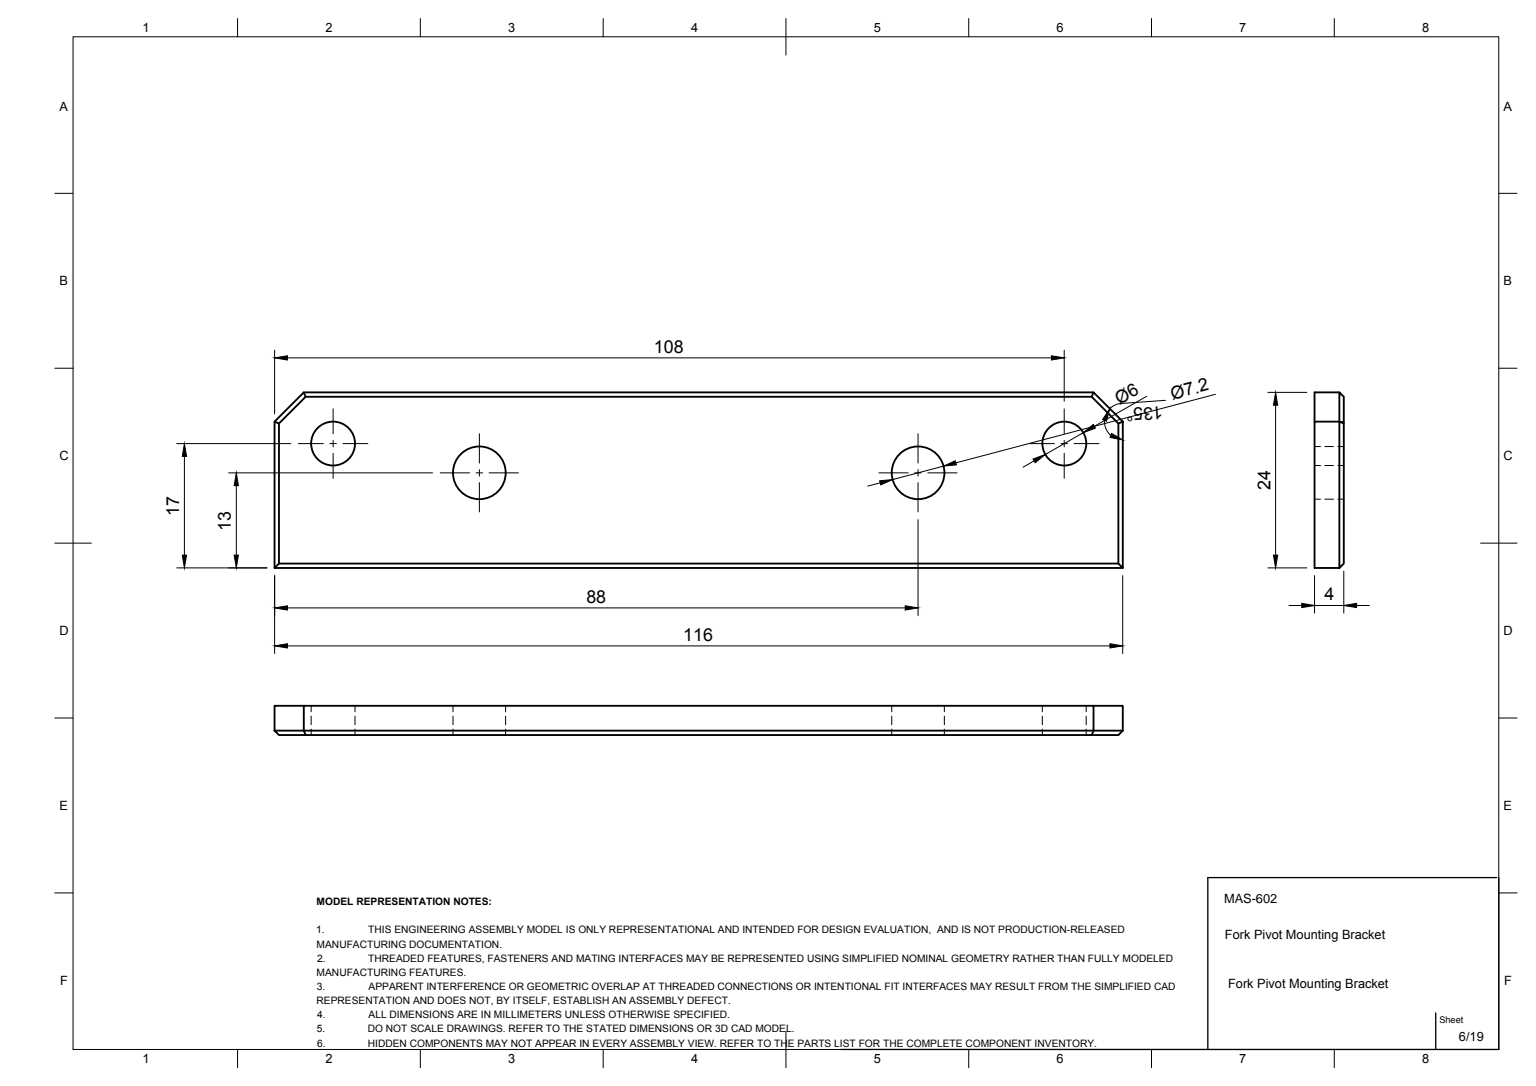
ISO-10303-21;
HEADER;
/* Generated by software containing ST-Developer
 * from STEP Tools, Inc. (www.steptools.com) 
 */

FILE_DESCRIPTION(
/* description */ (''),
/* implementation_level */ '2;1');

FILE_NAME(
/* name */ 'Fork Pivot Mounting Bracket.step',
/* time_stamp */ '2026-10-15T14:42:47-07:00',
/* author */ (''),
/* organization */ (''),
/* preprocessor_version */ 'ST-DEVELOPER v20.2',
/* originating_system */ 'Autodesk Translation Framework v15.15.0.0',
/* authorisation */ '');

FILE_SCHEMA (('AUTOMOTIVE_DESIGN { 1 0 10303 214 3 1 1 }'));
ENDSEC;

DATA;
#10=MECHANICAL_DESIGN_GEOMETRIC_PRESENTATION_REPRESENTATION('',(#237),#85789);
#201=SHAPE_REPRESENTATION_RELATIONSHIP('SRR','None',#85866,#219);
#219=ADVANCED_BREP_SHAPE_REPRESENTATION('',(#255),#85774);
#237=STYLED_ITEM('',(#85965),#255);
#255=MANIFOLD_SOLID_BREP('Body1',#9884);
#429=FACE_BOUND('',#3202,.T.);
#430=FACE_BOUND('',#3203,.T.);
#431=FACE_BOUND('',#3204,.T.);
#432=FACE_BOUND('',#3205,.T.);
#433=FACE_BOUND('',#3214,.T.);
#434=FACE_BOUND('',#3215,.T.);
#435=FACE_BOUND('',#3216,.T.);
#436=FACE_BOUND('',#3217,.T.);
#1066=PLANE('',#10454);
#1067=PLANE('',#10455);
#1068=PLANE('',#10456);
#1069=PLANE('',#10457);
#1070=PLANE('',#10458);
#1071=PLANE('',#10459);
#1072=PLANE('',#10460);
#1073=PLANE('',#10461);
#1074=PLANE('',#10462);
#1075=PLANE('',#10463);
#1076=PLANE('',#10476);
#1077=PLANE('',#10477);
#1078=PLANE('',#10478);
#1079=PLANE('',#10479);
#1435=LINE('',#23809,#1971);
#1436=LINE('',#23811,#1972);
#1437=LINE('',#23813,#1973);
#1438=LINE('',#23814,#1974);
#1439=LINE('',#23817,#1975);
#1440=LINE('',#23819,#1976);
#1441=LINE('',#23820,#1977);
#1442=LINE('',#23823,#1978);
#1443=LINE('',#23825,#1979);
#1444=LINE('',#23826,#1980);
#1445=LINE('',#23829,#1981);
#1446=LINE('',#23831,#1982);
#1447=LINE('',#23832,#1983);
#1448=LINE('',#23835,#1984);
#1449=LINE('',#23837,#1985);
#1450=LINE('',#23838,#1986);
#1451=LINE('',#23840,#1987);
#1452=LINE('',#23841,#1988);
#1453=LINE('',#23844,#1989);
#1454=LINE('',#23846,#1990);
#1455=LINE('',#23847,#1991);
#1456=LINE('',#23850,#1992);
#1457=LINE('',#23851,#1993);
#1458=LINE('',#23854,#1994);
#1459=LINE('',#23855,#1995);
#1460=LINE('',#23868,#1996);
#1461=LINE('',#23872,#1997);
#1462=LINE('',#23876,#1998);
#1463=LINE('',#23880,#1999);
#1464=LINE('',#23883,#2000);
#1465=LINE('',#23884,#2001);
#1466=LINE('',#23887,#2002);
#1467=LINE('',#23888,#2003);
#1468=LINE('',#23890,#2004);
#1971=VECTOR('',#11909,1.);
#1972=VECTOR('',#11910,1.);
#1973=VECTOR('',#11911,1.);
#1974=VECTOR('',#11912,1.);
#1975=VECTOR('',#11915,1.);
#1976=VECTOR('',#11916,1.);
#1977=VECTOR('',#11917,1.);
#1978=VECTOR('',#11920,1.);
#1979=VECTOR('',#11921,1.);
#1980=VECTOR('',#11922,1.);
#1981=VECTOR('',#11925,1.);
#1982=VECTOR('',#11926,1.);
#1983=VECTOR('',#11927,1.);
#1984=VECTOR('',#11930,1.);
#1985=VECTOR('',#11931,1.);
#1986=VECTOR('',#11932,1.);
#1987=VECTOR('',#11935,1.);
#1988=VECTOR('',#11936,1.);
#1989=VECTOR('',#11939,1.);
#1990=VECTOR('',#11940,1.);
#1991=VECTOR('',#11941,1.);
#1992=VECTOR('',#11944,1.);
#1993=VECTOR('',#11945,1.);
#1994=VECTOR('',#11948,1.);
#1995=VECTOR('',#11949,1.);
#1996=VECTOR('',#11964,0.36);
#1997=VECTOR('',#11969,0.3);
#1998=VECTOR('',#11974,0.3);
#1999=VECTOR('',#11979,0.36);
#2000=VECTOR('',#11982,1.);
#2001=VECTOR('',#11983,1.);
#2002=VECTOR('',#11986,1.);
#2003=VECTOR('',#11987,1.);
#2004=VECTOR('',#11990,1.);
#2322=CYLINDRICAL_SURFACE('',#10468,0.36);
#2323=CYLINDRICAL_SURFACE('',#10470,0.3);
#2324=CYLINDRICAL_SURFACE('',#10472,0.3);
#2325=CYLINDRICAL_SURFACE('',#10474,0.36);
#2648=FACE_OUTER_BOUND('',#3192,.T.);
#2649=FACE_OUTER_BOUND('',#3193,.T.);
#2650=FACE_OUTER_BOUND('',#3194,.T.);
#2651=FACE_OUTER_BOUND('',#3195,.T.);
#2652=FACE_OUTER_BOUND('',#3196,.T.);
#2653=FACE_OUTER_BOUND('',#3197,.T.);
#2654=FACE_OUTER_BOUND('',#3198,.T.);
#2655=FACE_OUTER_BOUND('',#3199,.T.);
#2656=FACE_OUTER_BOUND('',#3200,.T.);
#2657=FACE_OUTER_BOUND('',#3201,.T.);
#2658=FACE_OUTER_BOUND('',#3206,.T.);
#2659=FACE_OUTER_BOUND('',#3207,.T.);
#2660=FACE_OUTER_BOUND('',#3208,.T.);
#2661=FACE_OUTER_BOUND('',#3209,.T.);
#2662=FACE_OUTER_BOUND('',#3210,.T.);
#2663=FACE_OUTER_BOUND('',#3211,.T.);
#2664=FACE_OUTER_BOUND('',#3212,.T.);
#2665=FACE_OUTER_BOUND('',#3213,.T.);
#3192=EDGE_LOOP('',(#7641,#7642,#7643,#7644));
#3193=EDGE_LOOP('',(#7645,#7646,#7647,#7648));
#3194=EDGE_LOOP('',(#7649,#7650,#7651,#7652));
#3195=EDGE_LOOP('',(#7653,#7654,#7655,#7656));
#3196=EDGE_LOOP('',(#7657,#7658,#7659,#7660));
#3197=EDGE_LOOP('',(#7661,#7662,#7663,#7664));
#3198=EDGE_LOOP('',(#7665,#7666,#7667,#7668));
#3199=EDGE_LOOP('',(#7669,#7670,#7671,#7672));
#3200=EDGE_LOOP('',(#7673,#7674,#7675,#7676));
#3201=EDGE_LOOP('',(#7677,#7678,#7679,#7680,#7681,#7682));
#3202=EDGE_LOOP('',(#7683));
#3203=EDGE_LOOP('',(#7684));
#3204=EDGE_LOOP('',(#7685));
#3205=EDGE_LOOP('',(#7686));
#3206=EDGE_LOOP('',(#7687,#7688,#7689,#7690));
#3207=EDGE_LOOP('',(#7691,#7692,#7693,#7694));
#3208=EDGE_LOOP('',(#7695,#7696,#7697,#7698));
#3209=EDGE_LOOP('',(#7699,#7700,#7701,#7702));
#3210=EDGE_LOOP('',(#7703,#7704,#7705,#7706));
#3211=EDGE_LOOP('',(#7707,#7708,#7709,#7710));
#3212=EDGE_LOOP('',(#7711,#7712,#7713,#7714));
#3213=EDGE_LOOP('',(#7715,#7716,#7717,#7718,#7719,#7720));
#3214=EDGE_LOOP('',(#7721));
#3215=EDGE_LOOP('',(#7722));
#3216=EDGE_LOOP('',(#7723));
#3217=EDGE_LOOP('',(#7724));
#3684=CIRCLE('',#10464,0.36);
#3685=CIRCLE('',#10465,0.3);
#3686=CIRCLE('',#10466,0.3);
#3687=CIRCLE('',#10467,0.36);
#3688=CIRCLE('',#10469,0.36);
#3689=CIRCLE('',#10471,0.3);
#3690=CIRCLE('',#10473,0.3);
#3691=CIRCLE('',#10475,0.36);
#4275=VERTEX_POINT('',#23807);
#4276=VERTEX_POINT('',#23808);
#4277=VERTEX_POINT('',#23810);
#4278=VERTEX_POINT('',#23812);
#4279=VERTEX_POINT('',#23816);
#4280=VERTEX_POINT('',#23818);
#4281=VERTEX_POINT('',#23822);
#4282=VERTEX_POINT('',#23824);
#4283=VERTEX_POINT('',#23828);
#4284=VERTEX_POINT('',#23830);
#4285=VERTEX_POINT('',#23834);
#4286=VERTEX_POINT('',#23836);
#4287=VERTEX_POINT('',#23843);
#4288=VERTEX_POINT('',#23845);
#4289=VERTEX_POINT('',#23849);
#4290=VERTEX_POINT('',#23853);
#4291=VERTEX_POINT('',#23857);
#4292=VERTEX_POINT('',#23859);
#4293=VERTEX_POINT('',#23861);
#4294=VERTEX_POINT('',#23863);
#4295=VERTEX_POINT('',#23866);
#4296=VERTEX_POINT('',#23870);
#4297=VERTEX_POINT('',#23874);
#4298=VERTEX_POINT('',#23878);
#4299=VERTEX_POINT('',#23882);
#4300=VERTEX_POINT('',#23886);
#5548=EDGE_CURVE('',#4275,#4276,#1435,.T.);
#5549=EDGE_CURVE('',#4276,#4277,#1436,.T.);
#5550=EDGE_CURVE('',#4277,#4278,#1437,.T.);
#5551=EDGE_CURVE('',#4275,#4278,#1438,.T.);
#5552=EDGE_CURVE('',#4276,#4279,#1439,.T.);
#5553=EDGE_CURVE('',#4279,#4280,#1440,.T.);
#5554=EDGE_CURVE('',#4280,#4277,#1441,.T.);
#5555=EDGE_CURVE('',#4279,#4281,#1442,.T.);
#5556=EDGE_CURVE('',#4281,#4282,#1443,.T.);
#5557=EDGE_CURVE('',#4282,#4280,#1444,.T.);
#5558=EDGE_CURVE('',#4281,#4283,#1445,.T.);
#5559=EDGE_CURVE('',#4283,#4284,#1446,.T.);
#5560=EDGE_CURVE('',#4284,#4282,#1447,.T.);
#5561=EDGE_CURVE('',#4285,#4284,#1448,.T.);
#5562=EDGE_CURVE('',#4283,#4286,#1449,.T.);
#5563=EDGE_CURVE('',#4286,#4285,#1450,.T.);
#5564=EDGE_CURVE('',#4278,#4285,#1451,.T.);
#5565=EDGE_CURVE('',#4286,#4275,#1452,.T.);
#5566=EDGE_CURVE('',#4287,#4285,#1453,.T.);
#5567=EDGE_CURVE('',#4287,#4288,#1454,.T.);
#5568=EDGE_CURVE('',#4288,#4284,#1455,.T.);
#5569=EDGE_CURVE('',#4289,#4278,#1456,.T.);
#5570=EDGE_CURVE('',#4289,#4287,#1457,.T.);
#5571=EDGE_CURVE('',#4290,#4277,#1458,.T.);
#5572=EDGE_CURVE('',#4290,#4289,#1459,.T.);
#5573=EDGE_CURVE('',#4291,#4291,#3684,.T.);
#5574=EDGE_CURVE('',#4292,#4292,#3685,.T.);
#5575=EDGE_CURVE('',#4293,#4293,#3686,.T.);
#5576=EDGE_CURVE('',#4294,#4294,#3687,.T.);
#5577=EDGE_CURVE('',#4295,#4295,#3688,.T.);
#5578=EDGE_CURVE('',#4295,#4294,#1460,.T.);
#5579=EDGE_CURVE('',#4296,#4296,#3689,.T.);
#5580=EDGE_CURVE('',#4296,#4293,#1461,.T.);
#5581=EDGE_CURVE('',#4297,#4297,#3690,.T.);
#5582=EDGE_CURVE('',#4297,#4292,#1462,.T.);
#5583=EDGE_CURVE('',#4298,#4298,#3691,.T.);
#5584=EDGE_CURVE('',#4298,#4291,#1463,.T.);
#5585=EDGE_CURVE('',#4299,#4280,#1464,.T.);
#5586=EDGE_CURVE('',#4299,#4290,#1465,.T.);
#5587=EDGE_CURVE('',#4300,#4282,#1466,.T.);
#5588=EDGE_CURVE('',#4300,#4299,#1467,.T.);
#5589=EDGE_CURVE('',#4288,#4300,#1468,.T.);
#7641=ORIENTED_EDGE('',*,*,#5548,.T.);
#7642=ORIENTED_EDGE('',*,*,#5549,.T.);
#7643=ORIENTED_EDGE('',*,*,#5550,.T.);
#7644=ORIENTED_EDGE('',*,*,#5551,.F.);
#7645=ORIENTED_EDGE('',*,*,#5552,.T.);
#7646=ORIENTED_EDGE('',*,*,#5553,.T.);
#7647=ORIENTED_EDGE('',*,*,#5554,.T.);
#7648=ORIENTED_EDGE('',*,*,#5549,.F.);
#7649=ORIENTED_EDGE('',*,*,#5555,.T.);
#7650=ORIENTED_EDGE('',*,*,#5556,.T.);
#7651=ORIENTED_EDGE('',*,*,#5557,.T.);
#7652=ORIENTED_EDGE('',*,*,#5553,.F.);
#7653=ORIENTED_EDGE('',*,*,#5558,.T.);
#7654=ORIENTED_EDGE('',*,*,#5559,.T.);
#7655=ORIENTED_EDGE('',*,*,#5560,.T.);
#7656=ORIENTED_EDGE('',*,*,#5556,.F.);
#7657=ORIENTED_EDGE('',*,*,#5561,.T.);
#7658=ORIENTED_EDGE('',*,*,#5559,.F.);
#7659=ORIENTED_EDGE('',*,*,#5562,.T.);
#7660=ORIENTED_EDGE('',*,*,#5563,.T.);
#7661=ORIENTED_EDGE('',*,*,#5564,.T.);
#7662=ORIENTED_EDGE('',*,*,#5563,.F.);
#7663=ORIENTED_EDGE('',*,*,#5565,.T.);
#7664=ORIENTED_EDGE('',*,*,#5551,.T.);
#7665=ORIENTED_EDGE('',*,*,#5561,.F.);
#7666=ORIENTED_EDGE('',*,*,#5566,.F.);
#7667=ORIENTED_EDGE('',*,*,#5567,.T.);
#7668=ORIENTED_EDGE('',*,*,#5568,.T.);
#7669=ORIENTED_EDGE('',*,*,#5564,.F.);
#7670=ORIENTED_EDGE('',*,*,#5569,.F.);
#7671=ORIENTED_EDGE('',*,*,#5570,.T.);
#7672=ORIENTED_EDGE('',*,*,#5566,.T.);
#7673=ORIENTED_EDGE('',*,*,#5550,.F.);
#7674=ORIENTED_EDGE('',*,*,#5571,.F.);
#7675=ORIENTED_EDGE('',*,*,#5572,.T.);
#7676=ORIENTED_EDGE('',*,*,#5569,.T.);
#7677=ORIENTED_EDGE('',*,*,#5548,.F.);
#7678=ORIENTED_EDGE('',*,*,#5565,.F.);
#7679=ORIENTED_EDGE('',*,*,#5562,.F.);
#7680=ORIENTED_EDGE('',*,*,#5558,.F.);
#7681=ORIENTED_EDGE('',*,*,#5555,.F.);
#7682=ORIENTED_EDGE('',*,*,#5552,.F.);
#7683=ORIENTED_EDGE('',*,*,#5573,.T.);
#7684=ORIENTED_EDGE('',*,*,#5574,.T.);
#7685=ORIENTED_EDGE('',*,*,#5575,.T.);
#7686=ORIENTED_EDGE('',*,*,#5576,.T.);
#7687=ORIENTED_EDGE('',*,*,#5577,.F.);
#7688=ORIENTED_EDGE('',*,*,#5578,.T.);
#7689=ORIENTED_EDGE('',*,*,#5576,.F.);
#7690=ORIENTED_EDGE('',*,*,#5578,.F.);
#7691=ORIENTED_EDGE('',*,*,#5579,.F.);
#7692=ORIENTED_EDGE('',*,*,#5580,.T.);
#7693=ORIENTED_EDGE('',*,*,#5575,.F.);
#7694=ORIENTED_EDGE('',*,*,#5580,.F.);
#7695=ORIENTED_EDGE('',*,*,#5581,.F.);
#7696=ORIENTED_EDGE('',*,*,#5582,.T.);
#7697=ORIENTED_EDGE('',*,*,#5574,.F.);
#7698=ORIENTED_EDGE('',*,*,#5582,.F.);
#7699=ORIENTED_EDGE('',*,*,#5583,.F.);
#7700=ORIENTED_EDGE('',*,*,#5584,.T.);
#7701=ORIENTED_EDGE('',*,*,#5573,.F.);
#7702=ORIENTED_EDGE('',*,*,#5584,.F.);
#7703=ORIENTED_EDGE('',*,*,#5554,.F.);
#7704=ORIENTED_EDGE('',*,*,#5585,.F.);
#7705=ORIENTED_EDGE('',*,*,#5586,.T.);
#7706=ORIENTED_EDGE('',*,*,#5571,.T.);
#7707=ORIENTED_EDGE('',*,*,#5557,.F.);
#7708=ORIENTED_EDGE('',*,*,#5587,.F.);
#7709=ORIENTED_EDGE('',*,*,#5588,.T.);
#7710=ORIENTED_EDGE('',*,*,#5585,.T.);
#7711=ORIENTED_EDGE('',*,*,#5560,.F.);
#7712=ORIENTED_EDGE('',*,*,#5568,.F.);
#7713=ORIENTED_EDGE('',*,*,#5589,.T.);
#7714=ORIENTED_EDGE('',*,*,#5587,.T.);
#7715=ORIENTED_EDGE('',*,*,#5589,.F.);
#7716=ORIENTED_EDGE('',*,*,#5567,.F.);
#7717=ORIENTED_EDGE('',*,*,#5570,.F.);
#7718=ORIENTED_EDGE('',*,*,#5572,.F.);
#7719=ORIENTED_EDGE('',*,*,#5586,.F.);
#7720=ORIENTED_EDGE('',*,*,#5588,.F.);
#7721=ORIENTED_EDGE('',*,*,#5577,.T.);
#7722=ORIENTED_EDGE('',*,*,#5579,.T.);
#7723=ORIENTED_EDGE('',*,*,#5581,.T.);
#7724=ORIENTED_EDGE('',*,*,#5583,.T.);
#9626=ADVANCED_FACE('',(#2648),#1066,.T.);
#9627=ADVANCED_FACE('',(#2649),#1067,.T.);
#9628=ADVANCED_FACE('',(#2650),#1068,.T.);
#9629=ADVANCED_FACE('',(#2651),#1069,.T.);
#9630=ADVANCED_FACE('',(#2652),#1070,.T.);
#9631=ADVANCED_FACE('',(#2653),#1071,.T.);
#9632=ADVANCED_FACE('',(#2654),#1072,.T.);
#9633=ADVANCED_FACE('',(#2655),#1073,.T.);
#9634=ADVANCED_FACE('',(#2656),#1074,.T.);
#9635=ADVANCED_FACE('',(#2657,#429,#430,#431,#432),#1075,.T.);
#9636=ADVANCED_FACE('',(#2658),#2322,.F.);
#9637=ADVANCED_FACE('',(#2659),#2323,.F.);
#9638=ADVANCED_FACE('',(#2660),#2324,.F.);
#9639=ADVANCED_FACE('',(#2661),#2325,.F.);
#9640=ADVANCED_FACE('',(#2662),#1076,.T.);
#9641=ADVANCED_FACE('',(#2663),#1077,.T.);
#9642=ADVANCED_FACE('',(#2664),#1078,.T.);
#9643=ADVANCED_FACE('',(#2665,#433,#434,#435,#436),#1079,.T.);
#9884=CLOSED_SHELL('',(#9626,#9627,#9628,#9629,#9630,#9631,#9632,#9633,
#9634,#9635,#9636,#9637,#9638,#9639,#9640,#9641,#9642,#9643));
#10453=AXIS2_PLACEMENT_3D('',#23805,#11905,#11906);
#10454=AXIS2_PLACEMENT_3D('',#23806,#11907,#11908);
#10455=AXIS2_PLACEMENT_3D('',#23815,#11913,#11914);
#10456=AXIS2_PLACEMENT_3D('',#23821,#11918,#11919);
#10457=AXIS2_PLACEMENT_3D('',#23827,#11923,#11924);
#10458=AXIS2_PLACEMENT_3D('',#23833,#11928,#11929);
#10459=AXIS2_PLACEMENT_3D('',#23839,#11933,#11934);
#10460=AXIS2_PLACEMENT_3D('',#23842,#11937,#11938);
#10461=AXIS2_PLACEMENT_3D('',#23848,#11942,#11943);
#10462=AXIS2_PLACEMENT_3D('',#23852,#11946,#11947);
#10463=AXIS2_PLACEMENT_3D('',#23856,#11950,#11951);
#10464=AXIS2_PLACEMENT_3D('',#23858,#11952,#11953);
#10465=AXIS2_PLACEMENT_3D('',#23860,#11954,#11955);
#10466=AXIS2_PLACEMENT_3D('',#23862,#11956,#11957);
#10467=AXIS2_PLACEMENT_3D('',#23864,#11958,#11959);
#10468=AXIS2_PLACEMENT_3D('',#23865,#11960,#11961);
#10469=AXIS2_PLACEMENT_3D('',#23867,#11962,#11963);
#10470=AXIS2_PLACEMENT_3D('',#23869,#11965,#11966);
#10471=AXIS2_PLACEMENT_3D('',#23871,#11967,#11968);
#10472=AXIS2_PLACEMENT_3D('',#23873,#11970,#11971);
#10473=AXIS2_PLACEMENT_3D('',#23875,#11972,#11973);
#10474=AXIS2_PLACEMENT_3D('',#23877,#11975,#11976);
#10475=AXIS2_PLACEMENT_3D('',#23879,#11977,#11978);
#10476=AXIS2_PLACEMENT_3D('',#23881,#11980,#11981);
#10477=AXIS2_PLACEMENT_3D('',#23885,#11984,#11985);
#10478=AXIS2_PLACEMENT_3D('',#23889,#11988,#11989);
#10479=AXIS2_PLACEMENT_3D('',#23891,#11991,#11992);
#11905=DIRECTION('axis',(0.,0.,1.));
#11906=DIRECTION('refdir',(1.,0.,0.));
#11907=DIRECTION('center_axis',(0.70710678118655,-0.707106781186545,0.));
#11908=DIRECTION('ref_axis',(0.,0.,-1.));
#11909=DIRECTION('',(0.,0.,-1.));
#11910=DIRECTION('',(0.577350269189622,0.577350269189625,-0.57735026918963));
#11911=DIRECTION('',(0.,0.,1.));
#11912=DIRECTION('',(0.678598344545843,0.678598344545847,0.281084637714829));
#11913=DIRECTION('center_axis',(0.,-0.70710678118655,-0.707106781186545));
#11914=DIRECTION('ref_axis',(-1.,0.,0.));
#11915=DIRECTION('',(-1.,0.,0.));
#11916=DIRECTION('',(-0.577350269189622,0.577350269189625,-0.57735026918963));
#11917=DIRECTION('',(1.,0.,0.));
#11918=DIRECTION('center_axis',(-0.70710678118655,-0.707106781186545,0.));
#11919=DIRECTION('ref_axis',(0.,0.,1.));
#11920=DIRECTION('',(0.,0.,1.));
#11921=DIRECTION('',(-0.678598344545839,0.678598344545844,0.281084637714847));
#11922=DIRECTION('',(0.,0.,-1.));
#11923=DIRECTION('center_axis',(-0.499999999999994,-0.707106781186556,0.499999999999993));
#11924=DIRECTION('ref_axis',(0.707106781186547,-1.66533453693739E-16,0.707106781186548));
#11925=DIRECTION('',(0.707106781186547,0.,0.707106781186548));
#11926=DIRECTION('',(-0.281084637714836,0.678598344545841,0.678598344545847));
#11927=DIRECTION('',(-0.707106781186547,0.,-0.707106781186548));
#11928=DIRECTION('center_axis',(0.,-0.70710678118655,0.707106781186545));
#11929=DIRECTION('ref_axis',(1.,0.,0.));
#11930=DIRECTION('',(-1.,0.,0.));
#11931=DIRECTION('',(1.,0.,0.));
#11932=DIRECTION('',(0.281084637714827,0.678598344545843,0.678598344545848));
#11933=DIRECTION('center_axis',(0.499999999999997,-0.707106781186553,0.499999999999996));
#11934=DIRECTION('ref_axis',(0.707106781186547,1.66533453693763E-16,-0.707106781186548));
#11935=DIRECTION('',(-0.707106781186547,0.,0.707106781186548));
#11936=DIRECTION('',(0.707106781186547,0.,-0.707106781186548));
#11937=DIRECTION('center_axis',(0.,0.,1.));
#11938=DIRECTION('ref_axis',(-1.,0.,0.));
#11939=DIRECTION('',(0.,-1.,0.));
#11940=DIRECTION('',(-1.,0.,0.));
#11941=DIRECTION('',(0.,-1.,0.));
#11942=DIRECTION('center_axis',(0.707106781186548,0.,0.707106781186547));
#11943=DIRECTION('ref_axis',(-0.707106781186547,0.,0.707106781186548));
#11944=DIRECTION('',(0.,-1.,0.));
#11945=DIRECTION('',(-0.707106781186547,0.,0.707106781186548));
#11946=DIRECTION('center_axis',(1.,0.,0.));
#11947=DIRECTION('ref_axis',(0.,0.,1.));
#11948=DIRECTION('',(0.,-1.,0.));
#11949=DIRECTION('',(0.,0.,1.));
#11950=DIRECTION('center_axis',(0.,-1.,0.));
#11951=DIRECTION('ref_axis',(0.,0.,-1.));
#11952=DIRECTION('center_axis',(0.,1.,0.));
#11953=DIRECTION('ref_axis',(1.,0.,0.));
#11954=DIRECTION('center_axis',(0.,1.,0.));
#11955=DIRECTION('ref_axis',(1.,0.,0.));
#11956=DIRECTION('center_axis',(0.,1.,0.));
#11957=DIRECTION('ref_axis',(1.,0.,0.));
#11958=DIRECTION('center_axis',(0.,1.,0.));
#11959=DIRECTION('ref_axis',(1.,0.,0.));
#11960=DIRECTION('center_axis',(0.,-1.,0.));
#11961=DIRECTION('ref_axis',(1.,0.,0.));
#11962=DIRECTION('center_axis',(0.,-1.,0.));
#11963=DIRECTION('ref_axis',(1.,0.,0.));
#11964=DIRECTION('',(0.,-1.,0.));
#11965=DIRECTION('center_axis',(0.,-1.,0.));
#11966=DIRECTION('ref_axis',(1.,0.,0.));
#11967=DIRECTION('center_axis',(0.,-1.,0.));
#11968=DIRECTION('ref_axis',(1.,0.,0.));
#11969=DIRECTION('',(0.,-1.,0.));
#11970=DIRECTION('center_axis',(0.,-1.,0.));
#11971=DIRECTION('ref_axis',(1.,0.,0.));
#11972=DIRECTION('center_axis',(0.,-1.,0.));
#11973=DIRECTION('ref_axis',(1.,0.,0.));
#11974=DIRECTION('',(0.,-1.,0.));
#11975=DIRECTION('center_axis',(0.,-1.,0.));
#11976=DIRECTION('ref_axis',(1.,0.,0.));
#11977=DIRECTION('center_axis',(0.,-1.,0.));
#11978=DIRECTION('ref_axis',(1.,0.,0.));
#11979=DIRECTION('',(0.,-1.,0.));
#11980=DIRECTION('center_axis',(0.,0.,-1.));
#11981=DIRECTION('ref_axis',(1.,0.,0.));
#11982=DIRECTION('',(0.,-1.,0.));
#11983=DIRECTION('',(1.,0.,0.));
#11984=DIRECTION('center_axis',(-1.,0.,0.));
#11985=DIRECTION('ref_axis',(0.,0.,-1.));
#11986=DIRECTION('',(0.,-1.,0.));
#11987=DIRECTION('',(0.,0.,-1.));
#11988=DIRECTION('center_axis',(-0.707106781186548,0.,0.707106781186547));
#11989=DIRECTION('ref_axis',(-0.707106781186547,0.,-0.707106781186548));
#11990=DIRECTION('',(-0.707106781186547,0.,-0.707106781186548));
#11991=DIRECTION('center_axis',(0.,1.,0.));
#11992=DIRECTION('ref_axis',(1.,0.,0.));
#23805=CARTESIAN_POINT('',(0.,0.,0.));
#23806=CARTESIAN_POINT('Origin',(5.77,-0.37,11.));
#23807=CARTESIAN_POINT('',(5.74,-0.4,12.3751471862576));
#23808=CARTESIAN_POINT('',(5.74,-0.4,10.46));
#23809=CARTESIAN_POINT('',(5.74,-0.4,11.));
#23810=CARTESIAN_POINT('',(5.8,-0.34,10.4));
#23811=CARTESIAN_POINT('',(5.74,-0.4,10.46));
#23812=CARTESIAN_POINT('',(5.8,-0.34,12.4));
#23813=CARTESIAN_POINT('',(5.8,-0.34,11.));
#23814=CARTESIAN_POINT('',(5.74,-0.4,12.3751471862576));
#23815=CARTESIAN_POINT('Origin',(-2.9,-0.37,10.43));
#23816=CARTESIAN_POINT('',(-5.74,-0.4,10.46));
#23817=CARTESIAN_POINT('',(-2.9,-0.4,10.46));
#23818=CARTESIAN_POINT('',(-5.8,-0.34,10.4));
#23819=CARTESIAN_POINT('',(-5.74,-0.4,10.46));
#23820=CARTESIAN_POINT('',(-2.9,-0.34,10.4));
#23821=CARTESIAN_POINT('Origin',(-5.77,-0.37,12.));
#23822=CARTESIAN_POINT('',(-5.74,-0.4,12.3751471862576));
#23823=CARTESIAN_POINT('',(-5.74,-0.4,12.));
#23824=CARTESIAN_POINT('',(-5.8,-0.34,12.4));
#23825=CARTESIAN_POINT('',(-5.74,-0.4,12.3751471862576));
#23826=CARTESIAN_POINT('',(-5.8,-0.34,12.));
#23827=CARTESIAN_POINT('Origin',(-4.32878679656441,-0.37,13.8287867965644));
#23828=CARTESIAN_POINT('',(-5.37514718625761,-0.4,12.74));
#23829=CARTESIAN_POINT('',(-4.30757359312881,-0.4,13.8075735931288));
#23830=CARTESIAN_POINT('',(-5.4,-0.34,12.8));
#23831=CARTESIAN_POINT('',(-5.37514718625761,-0.4,12.74));
#23832=CARTESIAN_POINT('',(-4.35,-0.34,13.85));
#23833=CARTESIAN_POINT('Origin',(2.7,-0.37,12.77));
#23834=CARTESIAN_POINT('',(5.4,-0.34,12.8));
#23835=CARTESIAN_POINT('',(2.7,-0.34,12.8));
#23836=CARTESIAN_POINT('',(5.37514718625761,-0.4,12.74));
#23837=CARTESIAN_POINT('',(2.7,-0.4,12.74));
#23838=CARTESIAN_POINT('',(5.37514718625761,-0.4,12.74));
#23839=CARTESIAN_POINT('Origin',(4.52878679656441,-0.37,13.6287867965644));
#23840=CARTESIAN_POINT('',(4.55,-0.34,13.65));
#23841=CARTESIAN_POINT('',(4.50757359312881,-0.4,13.6075735931288));
#23842=CARTESIAN_POINT('Origin',(5.4,0.,12.8));
#23843=CARTESIAN_POINT('',(5.4,0.,12.8));
#23844=CARTESIAN_POINT('',(5.4,0.,12.8));
#23845=CARTESIAN_POINT('',(-5.4,0.,12.8));
#23846=CARTESIAN_POINT('',(5.4,0.,12.8));
#23847=CARTESIAN_POINT('',(-5.4,0.,12.8));
#23848=CARTESIAN_POINT('Origin',(5.8,0.,12.4));
#23849=CARTESIAN_POINT('',(5.8,0.,12.4));
#23850=CARTESIAN_POINT('',(5.8,0.,12.4));
#23851=CARTESIAN_POINT('',(5.8,0.,12.4));
#23852=CARTESIAN_POINT('Origin',(5.8,0.,10.4));
#23853=CARTESIAN_POINT('',(5.8,0.,10.4));
#23854=CARTESIAN_POINT('',(5.8,0.,10.4));
#23855=CARTESIAN_POINT('',(5.8,0.,10.4));
#23856=CARTESIAN_POINT('Origin',(0.,-0.4,11.6));
#23857=CARTESIAN_POINT('',(-3.36,-0.4,11.7));
#23858=CARTESIAN_POINT('Origin',(-3.,-0.4,11.7));
#23859=CARTESIAN_POINT('',(4.7,-0.4,12.1));
#23860=CARTESIAN_POINT('Origin',(5.,-0.4,12.1));
#23861=CARTESIAN_POINT('',(-5.3,-0.4,12.1));
#23862=CARTESIAN_POINT('Origin',(-5.,-0.4,12.1));
#23863=CARTESIAN_POINT('',(2.64,-0.4,11.7));
#23864=CARTESIAN_POINT('Origin',(3.,-0.4,11.7));
#23865=CARTESIAN_POINT('Origin',(3.,0.,11.7));
#23866=CARTESIAN_POINT('',(2.64,0.,11.7));
#23867=CARTESIAN_POINT('Origin',(3.,0.,11.7));
#23868=CARTESIAN_POINT('',(2.64,0.,11.7));
#23869=CARTESIAN_POINT('Origin',(-5.,0.,12.1));
#23870=CARTESIAN_POINT('',(-5.3,0.,12.1));
#23871=CARTESIAN_POINT('Origin',(-5.,0.,12.1));
#23872=CARTESIAN_POINT('',(-5.3,0.,12.1));
#23873=CARTESIAN_POINT('Origin',(5.,0.,12.1));
#23874=CARTESIAN_POINT('',(4.7,0.,12.1));
#23875=CARTESIAN_POINT('Origin',(5.,0.,12.1));
#23876=CARTESIAN_POINT('',(4.7,0.,12.1));
#23877=CARTESIAN_POINT('Origin',(-3.,0.,11.7));
#23878=CARTESIAN_POINT('',(-3.36,0.,11.7));
#23879=CARTESIAN_POINT('Origin',(-3.,0.,11.7));
#23880=CARTESIAN_POINT('',(-3.36,0.,11.7));
#23881=CARTESIAN_POINT('Origin',(-5.8,0.,10.4));
#23882=CARTESIAN_POINT('',(-5.8,0.,10.4));
#23883=CARTESIAN_POINT('',(-5.8,0.,10.4));
#23884=CARTESIAN_POINT('',(-5.8,0.,10.4));
#23885=CARTESIAN_POINT('Origin',(-5.8,0.,12.4));
#23886=CARTESIAN_POINT('',(-5.8,0.,12.4));
#23887=CARTESIAN_POINT('',(-5.8,0.,12.4));
#23888=CARTESIAN_POINT('',(-5.8,0.,12.4));
#23889=CARTESIAN_POINT('Origin',(-5.4,0.,12.8));
#23890=CARTESIAN_POINT('',(-5.4,0.,12.8));
#23891=CARTESIAN_POINT('Origin',(0.,0.,11.6));
#85754=UNCERTAINTY_MEASURE_WITH_UNIT(LENGTH_MEASURE(0.001),#85790,
'DISTANCE_ACCURACY_VALUE',
'Maximum model space distance between geometric entities at asserted c
onnectivities');
#85769=UNCERTAINTY_MEASURE_WITH_UNIT(LENGTH_MEASURE(0.001),#85790,
'DISTANCE_ACCURACY_VALUE',
'Maximum model space distance between geometric entities at asserted c
onnectivities');
#85774=(
GEOMETRIC_REPRESENTATION_CONTEXT(3)
GLOBAL_UNCERTAINTY_ASSIGNED_CONTEXT((#85754))
GLOBAL_UNIT_ASSIGNED_CONTEXT((#85790,#85792,#85793))
REPRESENTATION_CONTEXT('','3D')
);
#85789=(
GEOMETRIC_REPRESENTATION_CONTEXT(3)
GLOBAL_UNCERTAINTY_ASSIGNED_CONTEXT((#85769))
GLOBAL_UNIT_ASSIGNED_CONTEXT((#85790,#85792,#85793))
REPRESENTATION_CONTEXT('','3D')
);
#85790=(
LENGTH_UNIT()
NAMED_UNIT(*)
SI_UNIT(.CENTI.,.METRE.)
);
#85792=(
NAMED_UNIT(*)
PLANE_ANGLE_UNIT()
SI_UNIT($,.RADIAN.)
);
#85793=(
NAMED_UNIT(*)
SI_UNIT($,.STERADIAN.)
SOLID_ANGLE_UNIT()
);
#85798=SHAPE_DEFINITION_REPRESENTATION(#85817,#85866);
#85817=PRODUCT_DEFINITION_SHAPE('',$,#85886);
#85866=SHAPE_REPRESENTATION('',(#10453),#85774);
#85881=PRODUCT_DEFINITION_CONTEXT('part definition',#85940,'design');
#85886=PRODUCT_DEFINITION('Fork Pivot Mounting Bracket',
'Fork Pivot Mounting Bracket',#85905,#85881);
#85905=PRODUCT_DEFINITION_FORMATION('',$,#85946);
#85940=APPLICATION_CONTEXT(
'Core Data for Automotive Mechanical Design Process');
#85941=PRODUCT_CONTEXT('part definition',#85940,'mechanical');
#85946=PRODUCT('Fork Pivot Mounting Bracket',
'Fork Pivot Mounting Bracket',$,(#85941));
#85965=PRESENTATION_STYLE_ASSIGNMENT((#85983));
#85983=SURFACE_STYLE_USAGE(.BOTH.,#86001);
#86001=SURFACE_SIDE_STYLE('',(#86019));
#86019=SURFACE_STYLE_FILL_AREA(#86037);
#86037=FILL_AREA_STYLE('Opaque(150,153,157)',(#86055));
#86055=FILL_AREA_STYLE_COLOUR('Opaque(150,153,157)',#86073);
#86073=COLOUR_RGB('Opaque(150,153,157)', 0.72549020, 0.75294118, 0.79215686);
ENDSEC;
END-ISO-10303-21;
